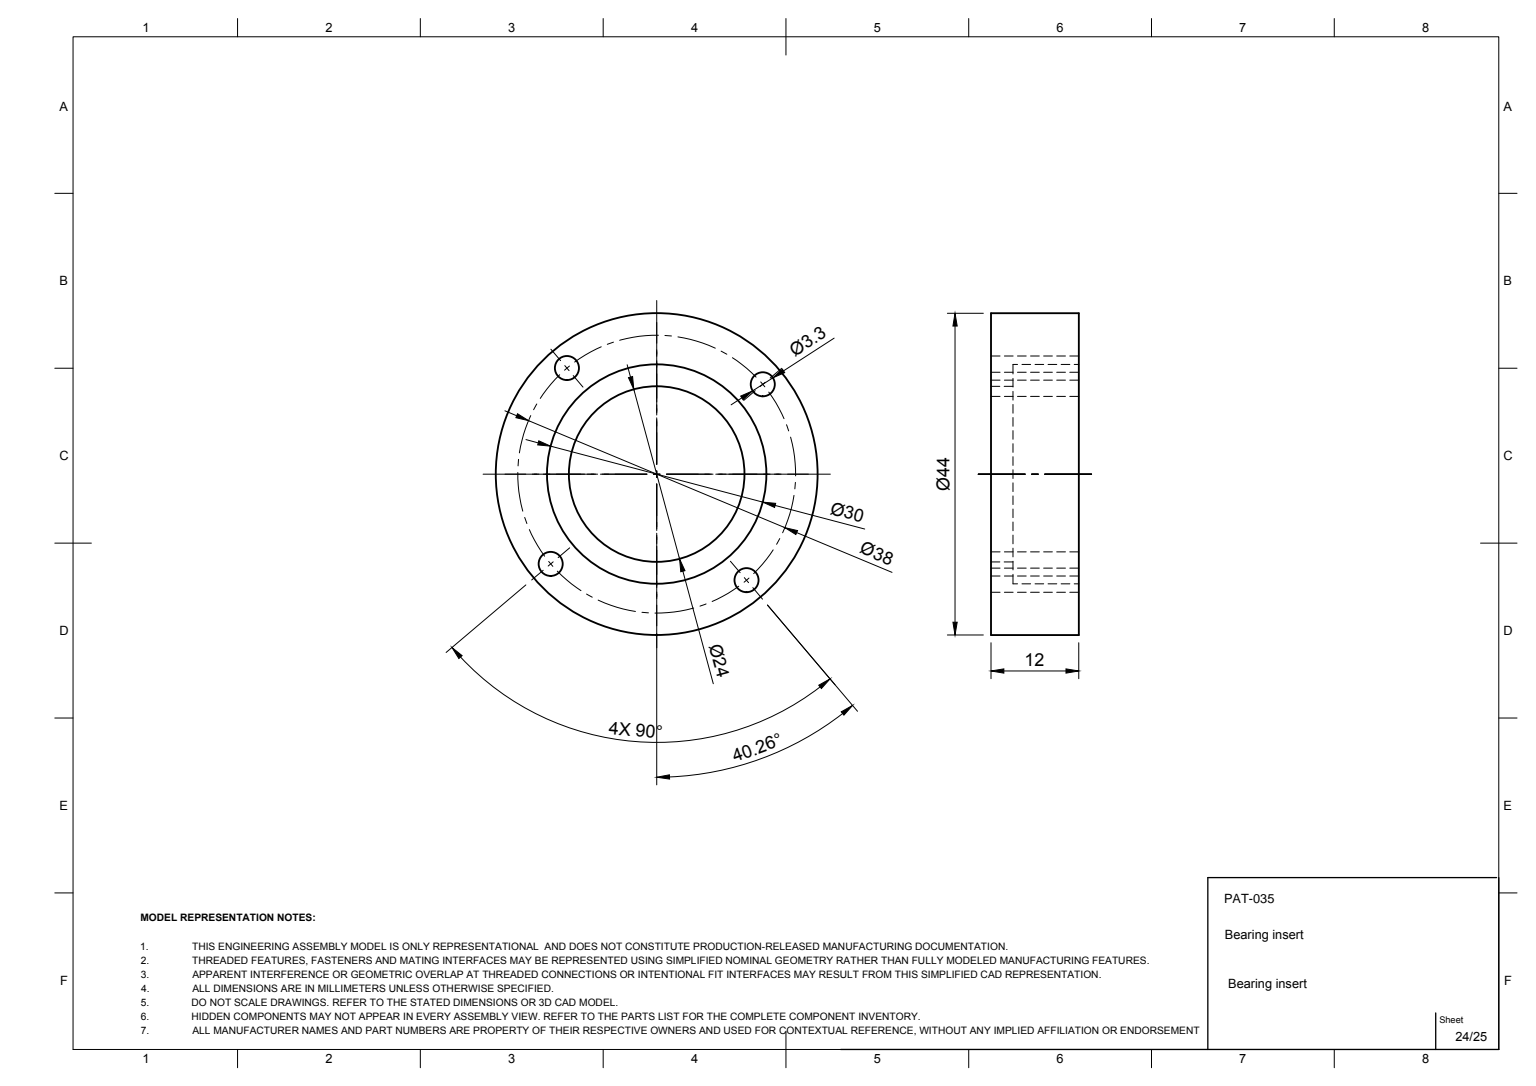
ISO-10303-21;
HEADER;
/* Generated by software containing ST-Developer
 * from STEP Tools, Inc. (www.steptools.com) 
 */

FILE_DESCRIPTION(
/* description */ ('Five-roller gravity conveyor'),
/* implementation_level */ '2;1');

FILE_NAME(
/* name */ 'Bearing insert.step',
/* time_stamp */ '2026-10-29T15:36:43-07:00',
/* author */ (''),
/* organization */ (''),
/* preprocessor_version */ 'ST-DEVELOPER v20.2',
/* originating_system */ 'Autodesk Translation Framework v15.17.0.0',
/* authorisation */ '');

FILE_SCHEMA (('AUTOMOTIVE_DESIGN { 1 0 10303 214 3 1 1 }'));
ENDSEC;

DATA;
#10=MECHANICAL_DESIGN_GEOMETRIC_PRESENTATION_REPRESENTATION('',(#335),#7806);
#291=SHAPE_REPRESENTATION_RELATIONSHIP('SRR','None',#7930,#309);
#309=ADVANCED_BREP_SHAPE_REPRESENTATION('',(#360),#7803);
#335=STYLED_ITEM('',(#8091),#360);
#360=MANIFOLD_SOLID_BREP('Body1',#4223);
#399=FACE_BOUND('',#1124,.T.);
#400=FACE_BOUND('',#1128,.T.);
#401=FACE_BOUND('',#1129,.T.);
#402=FACE_BOUND('',#1130,.T.);
#403=FACE_BOUND('',#1131,.T.);
#404=FACE_BOUND('',#1132,.T.);
#405=FACE_BOUND('',#1134,.T.);
#406=FACE_BOUND('',#1135,.T.);
#407=FACE_BOUND('',#1136,.T.);
#408=FACE_BOUND('',#1137,.T.);
#409=FACE_BOUND('',#1138,.T.);
#560=CIRCLE('',#4791,0.165);
#561=CIRCLE('',#4792,0.165);
#562=CIRCLE('',#4794,0.165);
#563=CIRCLE('',#4795,0.165);
#564=CIRCLE('',#4797,0.165);
#565=CIRCLE('',#4798,0.165);
#566=CIRCLE('',#4800,0.165);
#567=CIRCLE('',#4801,0.165);
#568=CIRCLE('',#4803,1.2);
#569=CIRCLE('',#4804,1.2);
#570=CIRCLE('',#4806,1.5);
#571=CIRCLE('',#4808,1.5);
#572=CIRCLE('',#4810,2.2);
#573=CIRCLE('',#4811,2.2);
#637=CYLINDRICAL_SURFACE('',#4790,0.165);
#638=CYLINDRICAL_SURFACE('',#4793,0.165);
#639=CYLINDRICAL_SURFACE('',#4796,0.165);
#640=CYLINDRICAL_SURFACE('',#4799,0.165);
#641=CYLINDRICAL_SURFACE('',#4802,1.2);
#642=CYLINDRICAL_SURFACE('',#4807,1.5);
#643=CYLINDRICAL_SURFACE('',#4809,2.2);
#849=FACE_OUTER_BOUND('',#1118,.T.);
#850=FACE_OUTER_BOUND('',#1119,.T.);
#851=FACE_OUTER_BOUND('',#1120,.T.);
#852=FACE_OUTER_BOUND('',#1121,.T.);
#853=FACE_OUTER_BOUND('',#1122,.T.);
#854=FACE_OUTER_BOUND('',#1123,.T.);
#855=FACE_OUTER_BOUND('',#1125,.T.);
#856=FACE_OUTER_BOUND('',#1126,.T.);
#857=FACE_OUTER_BOUND('',#1127,.T.);
#858=FACE_OUTER_BOUND('',#1133,.T.);
#1118=EDGE_LOOP('',(#3680,#3681,#3682,#3683));
#1119=EDGE_LOOP('',(#3684,#3685,#3686,#3687));
#1120=EDGE_LOOP('',(#3688,#3689,#3690,#3691));
#1121=EDGE_LOOP('',(#3692,#3693,#3694,#3695));
#1122=EDGE_LOOP('',(#3696,#3697,#3698,#3699));
#1123=EDGE_LOOP('',(#3700));
#1124=EDGE_LOOP('',(#3701));
#1125=EDGE_LOOP('',(#3702,#3703,#3704,#3705));
#1126=EDGE_LOOP('',(#3706,#3707,#3708,#3709));
#1127=EDGE_LOOP('',(#3710));
#1128=EDGE_LOOP('',(#3711));
#1129=EDGE_LOOP('',(#3712));
#1130=EDGE_LOOP('',(#3713));
#1131=EDGE_LOOP('',(#3714));
#1132=EDGE_LOOP('',(#3715));
#1133=EDGE_LOOP('',(#3716));
#1134=EDGE_LOOP('',(#3717));
#1135=EDGE_LOOP('',(#3718));
#1136=EDGE_LOOP('',(#3719));
#1137=EDGE_LOOP('',(#3720));
#1138=EDGE_LOOP('',(#3721));
#1479=LINE('',#7561,#1820);
#1480=LINE('',#7567,#1821);
#1481=LINE('',#7573,#1822);
#1482=LINE('',#7579,#1823);
#1483=LINE('',#7585,#1824);
#1484=LINE('',#7592,#1825);
#1485=LINE('',#7598,#1826);
#1820=VECTOR('',#5945,0.165);
#1821=VECTOR('',#5952,0.165);
#1822=VECTOR('',#5959,0.165);
#1823=VECTOR('',#5966,0.165);
#1824=VECTOR('',#5973,1.2);
#1825=VECTOR('',#5982,1.5);
#1826=VECTOR('',#5989,2.2);
#2174=VERTEX_POINT('',#7558);
#2175=VERTEX_POINT('',#7560);
#2176=VERTEX_POINT('',#7564);
#2177=VERTEX_POINT('',#7566);
#2178=VERTEX_POINT('',#7570);
#2179=VERTEX_POINT('',#7572);
#2180=VERTEX_POINT('',#7576);
#2181=VERTEX_POINT('',#7578);
#2182=VERTEX_POINT('',#7582);
#2183=VERTEX_POINT('',#7584);
#2184=VERTEX_POINT('',#7588);
#2185=VERTEX_POINT('',#7591);
#2186=VERTEX_POINT('',#7595);
#2187=VERTEX_POINT('',#7597);
#2683=EDGE_CURVE('',#2174,#2174,#560,.T.);
#2684=EDGE_CURVE('',#2174,#2175,#1479,.T.);
#2685=EDGE_CURVE('',#2175,#2175,#561,.T.);
#2686=EDGE_CURVE('',#2176,#2176,#562,.T.);
#2687=EDGE_CURVE('',#2176,#2177,#1480,.T.);
#2688=EDGE_CURVE('',#2177,#2177,#563,.T.);
#2689=EDGE_CURVE('',#2178,#2178,#564,.T.);
#2690=EDGE_CURVE('',#2178,#2179,#1481,.T.);
#2691=EDGE_CURVE('',#2179,#2179,#565,.T.);
#2692=EDGE_CURVE('',#2180,#2180,#566,.T.);
#2693=EDGE_CURVE('',#2180,#2181,#1482,.T.);
#2694=EDGE_CURVE('',#2181,#2181,#567,.T.);
#2695=EDGE_CURVE('',#2182,#2182,#568,.T.);
#2696=EDGE_CURVE('',#2182,#2183,#1483,.T.);
#2697=EDGE_CURVE('',#2183,#2183,#569,.T.);
#2698=EDGE_CURVE('',#2184,#2184,#570,.T.);
#2699=EDGE_CURVE('',#2184,#2185,#1484,.T.);
#2700=EDGE_CURVE('',#2185,#2185,#571,.T.);
#2701=EDGE_CURVE('',#2186,#2186,#572,.T.);
#2702=EDGE_CURVE('',#2186,#2187,#1485,.T.);
#2703=EDGE_CURVE('',#2187,#2187,#573,.T.);
#3680=ORIENTED_EDGE('',*,*,#2683,.F.);
#3681=ORIENTED_EDGE('',*,*,#2684,.T.);
#3682=ORIENTED_EDGE('',*,*,#2685,.F.);
#3683=ORIENTED_EDGE('',*,*,#2684,.F.);
#3684=ORIENTED_EDGE('',*,*,#2686,.F.);
#3685=ORIENTED_EDGE('',*,*,#2687,.T.);
#3686=ORIENTED_EDGE('',*,*,#2688,.F.);
#3687=ORIENTED_EDGE('',*,*,#2687,.F.);
#3688=ORIENTED_EDGE('',*,*,#2689,.F.);
#3689=ORIENTED_EDGE('',*,*,#2690,.T.);
#3690=ORIENTED_EDGE('',*,*,#2691,.F.);
#3691=ORIENTED_EDGE('',*,*,#2690,.F.);
#3692=ORIENTED_EDGE('',*,*,#2692,.F.);
#3693=ORIENTED_EDGE('',*,*,#2693,.T.);
#3694=ORIENTED_EDGE('',*,*,#2694,.F.);
#3695=ORIENTED_EDGE('',*,*,#2693,.F.);
#3696=ORIENTED_EDGE('',*,*,#2695,.F.);
#3697=ORIENTED_EDGE('',*,*,#2696,.T.);
#3698=ORIENTED_EDGE('',*,*,#2697,.T.);
#3699=ORIENTED_EDGE('',*,*,#2696,.F.);
#3700=ORIENTED_EDGE('',*,*,#2698,.F.);
#3701=ORIENTED_EDGE('',*,*,#2697,.F.);
#3702=ORIENTED_EDGE('',*,*,#2698,.T.);
#3703=ORIENTED_EDGE('',*,*,#2699,.T.);
#3704=ORIENTED_EDGE('',*,*,#2700,.T.);
#3705=ORIENTED_EDGE('',*,*,#2699,.F.);
#3706=ORIENTED_EDGE('',*,*,#2701,.F.);
#3707=ORIENTED_EDGE('',*,*,#2702,.T.);
#3708=ORIENTED_EDGE('',*,*,#2703,.T.);
#3709=ORIENTED_EDGE('',*,*,#2702,.F.);
#3710=ORIENTED_EDGE('',*,*,#2701,.T.);
#3711=ORIENTED_EDGE('',*,*,#2695,.T.);
#3712=ORIENTED_EDGE('',*,*,#2694,.T.);
#3713=ORIENTED_EDGE('',*,*,#2691,.T.);
#3714=ORIENTED_EDGE('',*,*,#2688,.T.);
#3715=ORIENTED_EDGE('',*,*,#2685,.T.);
#3716=ORIENTED_EDGE('',*,*,#2703,.F.);
#3717=ORIENTED_EDGE('',*,*,#2700,.F.);
#3718=ORIENTED_EDGE('',*,*,#2692,.T.);
#3719=ORIENTED_EDGE('',*,*,#2689,.T.);
#3720=ORIENTED_EDGE('',*,*,#2686,.T.);
#3721=ORIENTED_EDGE('',*,*,#2683,.T.);
#3951=PLANE('',#4805);
#3952=PLANE('',#4812);
#3953=PLANE('',#4813);
#4164=ADVANCED_FACE('',(#849),#637,.F.);
#4165=ADVANCED_FACE('',(#850),#638,.F.);
#4166=ADVANCED_FACE('',(#851),#639,.F.);
#4167=ADVANCED_FACE('',(#852),#640,.F.);
#4168=ADVANCED_FACE('',(#853),#641,.F.);
#4169=ADVANCED_FACE('',(#854,#399),#3951,.F.);
#4170=ADVANCED_FACE('',(#855),#642,.F.);
#4171=ADVANCED_FACE('',(#856),#643,.T.);
#4172=ADVANCED_FACE('',(#857,#400,#401,#402,#403,#404),#3952,.T.);
#4173=ADVANCED_FACE('',(#858,#405,#406,#407,#408,#409),#3953,.F.);
#4223=CLOSED_SHELL('',(#4164,#4165,#4166,#4167,#4168,#4169,#4170,#4171,
#4172,#4173));
#4789=AXIS2_PLACEMENT_3D('',#7556,#5939,#5940);
#4790=AXIS2_PLACEMENT_3D('',#7557,#5941,#5942);
#4791=AXIS2_PLACEMENT_3D('',#7559,#5943,#5944);
#4792=AXIS2_PLACEMENT_3D('',#7562,#5946,#5947);
#4793=AXIS2_PLACEMENT_3D('',#7563,#5948,#5949);
#4794=AXIS2_PLACEMENT_3D('',#7565,#5950,#5951);
#4795=AXIS2_PLACEMENT_3D('',#7568,#5953,#5954);
#4796=AXIS2_PLACEMENT_3D('',#7569,#5955,#5956);
#4797=AXIS2_PLACEMENT_3D('',#7571,#5957,#5958);
#4798=AXIS2_PLACEMENT_3D('',#7574,#5960,#5961);
#4799=AXIS2_PLACEMENT_3D('',#7575,#5962,#5963);
#4800=AXIS2_PLACEMENT_3D('',#7577,#5964,#5965);
#4801=AXIS2_PLACEMENT_3D('',#7580,#5967,#5968);
#4802=AXIS2_PLACEMENT_3D('',#7581,#5969,#5970);
#4803=AXIS2_PLACEMENT_3D('',#7583,#5971,#5972);
#4804=AXIS2_PLACEMENT_3D('',#7586,#5974,#5975);
#4805=AXIS2_PLACEMENT_3D('',#7587,#5976,#5977);
#4806=AXIS2_PLACEMENT_3D('',#7589,#5978,#5979);
#4807=AXIS2_PLACEMENT_3D('',#7590,#5980,#5981);
#4808=AXIS2_PLACEMENT_3D('',#7593,#5983,#5984);
#4809=AXIS2_PLACEMENT_3D('',#7594,#5985,#5986);
#4810=AXIS2_PLACEMENT_3D('',#7596,#5987,#5988);
#4811=AXIS2_PLACEMENT_3D('',#7599,#5990,#5991);
#4812=AXIS2_PLACEMENT_3D('',#7600,#5992,#5993);
#4813=AXIS2_PLACEMENT_3D('',#7601,#5994,#5995);
#5939=DIRECTION('axis',(0.,0.,1.));
#5940=DIRECTION('refdir',(1.,0.,0.));
#5941=DIRECTION('center_axis',(0.,1.,0.));
#5942=DIRECTION('ref_axis',(1.,0.,0.));
#5943=DIRECTION('center_axis',(0.,1.,0.));
#5944=DIRECTION('ref_axis',(1.,0.,0.));
#5945=DIRECTION('',(0.,1.,0.));
#5946=DIRECTION('center_axis',(0.,-1.,0.));
#5947=DIRECTION('ref_axis',(1.,0.,0.));
#5948=DIRECTION('center_axis',(0.,1.,0.));
#5949=DIRECTION('ref_axis',(1.,0.,0.));
#5950=DIRECTION('center_axis',(0.,1.,0.));
#5951=DIRECTION('ref_axis',(1.,0.,0.));
#5952=DIRECTION('',(0.,1.,0.));
#5953=DIRECTION('center_axis',(0.,-1.,0.));
#5954=DIRECTION('ref_axis',(1.,0.,0.));
#5955=DIRECTION('center_axis',(0.,1.,0.));
#5956=DIRECTION('ref_axis',(1.,0.,0.));
#5957=DIRECTION('center_axis',(0.,1.,0.));
#5958=DIRECTION('ref_axis',(1.,0.,0.));
#5959=DIRECTION('',(0.,1.,0.));
#5960=DIRECTION('center_axis',(0.,-1.,0.));
#5961=DIRECTION('ref_axis',(1.,0.,0.));
#5962=DIRECTION('center_axis',(0.,1.,0.));
#5963=DIRECTION('ref_axis',(1.,0.,0.));
#5964=DIRECTION('center_axis',(0.,1.,0.));
#5965=DIRECTION('ref_axis',(1.,0.,0.));
#5966=DIRECTION('',(0.,1.,0.));
#5967=DIRECTION('center_axis',(0.,-1.,0.));
#5968=DIRECTION('ref_axis',(1.,0.,0.));
#5969=DIRECTION('center_axis',(0.,1.,0.));
#5970=DIRECTION('ref_axis',(1.,0.,0.));
#5971=DIRECTION('center_axis',(0.,-1.,0.));
#5972=DIRECTION('ref_axis',(1.,0.,0.));
#5973=DIRECTION('',(0.,-1.,0.));
#5974=DIRECTION('center_axis',(0.,-1.,0.));
#5975=DIRECTION('ref_axis',(1.,0.,0.));
#5976=DIRECTION('center_axis',(0.,1.,0.));
#5977=DIRECTION('ref_axis',(1.,0.,0.));
#5978=DIRECTION('center_axis',(0.,1.,0.));
#5979=DIRECTION('ref_axis',(1.,0.,0.));
#5980=DIRECTION('center_axis',(0.,1.,0.));
#5981=DIRECTION('ref_axis',(1.,0.,0.));
#5982=DIRECTION('',(0.,-1.,0.));
#5983=DIRECTION('center_axis',(0.,-1.,0.));
#5984=DIRECTION('ref_axis',(1.,0.,0.));
#5985=DIRECTION('center_axis',(0.,1.,0.));
#5986=DIRECTION('ref_axis',(1.,0.,0.));
#5987=DIRECTION('center_axis',(0.,1.,0.));
#5988=DIRECTION('ref_axis',(1.,0.,0.));
#5989=DIRECTION('',(0.,-1.,0.));
#5990=DIRECTION('center_axis',(0.,1.,0.));
#5991=DIRECTION('ref_axis',(1.,0.,0.));
#5992=DIRECTION('center_axis',(0.,1.,0.));
#5993=DIRECTION('ref_axis',(1.,0.,0.));
#5994=DIRECTION('center_axis',(0.,1.,0.));
#5995=DIRECTION('ref_axis',(1.,0.,0.));
#7556=CARTESIAN_POINT('',(0.,0.,0.));
#7557=CARTESIAN_POINT('Origin',(-1.9,-0.1,4.5));
#7558=CARTESIAN_POINT('',(-2.065,0.,4.5));
#7559=CARTESIAN_POINT('Origin',(-1.9,0.,4.5));
#7560=CARTESIAN_POINT('',(-2.065,1.2,4.5));
#7561=CARTESIAN_POINT('',(-2.065,-0.1,4.5));
#7562=CARTESIAN_POINT('Origin',(-1.9,1.2,4.5));
#7563=CARTESIAN_POINT('Origin',(1.16341445918999E-16,-0.1,6.4));
#7564=CARTESIAN_POINT('',(-0.165,0.,6.4));
#7565=CARTESIAN_POINT('Origin',(1.16341445918999E-16,0.,6.4));
#7566=CARTESIAN_POINT('',(-0.165,1.2,6.4));
#7567=CARTESIAN_POINT('',(-0.165,-0.1,6.4));
#7568=CARTESIAN_POINT('Origin',(1.16341445918999E-16,1.2,6.4));
#7569=CARTESIAN_POINT('Origin',(1.9,-0.1,4.5));
#7570=CARTESIAN_POINT('',(1.735,0.,4.5));
#7571=CARTESIAN_POINT('Origin',(1.9,0.,4.5));
#7572=CARTESIAN_POINT('',(1.735,1.2,4.5));
#7573=CARTESIAN_POINT('',(1.735,-0.1,4.5));
#7574=CARTESIAN_POINT('Origin',(1.9,1.2,4.5));
#7575=CARTESIAN_POINT('Origin',(-3.49024337756996E-16,-0.1,2.6));
#7576=CARTESIAN_POINT('',(-0.165,0.,2.6));
#7577=CARTESIAN_POINT('Origin',(-3.49024337756996E-16,0.,2.6));
#7578=CARTESIAN_POINT('',(-0.165,1.2,2.6));
#7579=CARTESIAN_POINT('',(-0.165,-0.1,2.6));
#7580=CARTESIAN_POINT('Origin',(-3.49024337756996E-16,1.2,2.6));
#7581=CARTESIAN_POINT('Origin',(0.,0.9,4.5));
#7582=CARTESIAN_POINT('',(-1.2,1.2,4.5));
#7583=CARTESIAN_POINT('Origin',(0.,1.2,4.5));
#7584=CARTESIAN_POINT('',(-1.2,0.9,4.5));
#7585=CARTESIAN_POINT('',(-1.2,0.9,4.5));
#7586=CARTESIAN_POINT('Origin',(0.,0.9,4.5));
#7587=CARTESIAN_POINT('Origin',(0.,0.9,4.5));
#7588=CARTESIAN_POINT('',(-1.5,0.9,4.5));
#7589=CARTESIAN_POINT('Origin',(0.,0.9,4.5));
#7590=CARTESIAN_POINT('Origin',(0.,0.,4.5));
#7591=CARTESIAN_POINT('',(-1.5,0.,4.5));
#7592=CARTESIAN_POINT('',(-1.5,0.,4.5));
#7593=CARTESIAN_POINT('Origin',(0.,0.,4.5));
#7594=CARTESIAN_POINT('Origin',(0.,0.,4.5));
#7595=CARTESIAN_POINT('',(-2.2,1.2,4.5));
#7596=CARTESIAN_POINT('Origin',(0.,1.2,4.5));
#7597=CARTESIAN_POINT('',(-2.2,0.,4.5));
#7598=CARTESIAN_POINT('',(-2.2,0.,4.5));
#7599=CARTESIAN_POINT('Origin',(0.,0.,4.5));
#7600=CARTESIAN_POINT('Origin',(0.,1.2,4.5));
#7601=CARTESIAN_POINT('Origin',(0.,0.,4.5));
#7779=UNCERTAINTY_MEASURE_WITH_UNIT(LENGTH_MEASURE(0.001),#7807,
'DISTANCE_ACCURACY_VALUE',
'Maximum model space distance between geometric entities at asserted c
onnectivities');
#7782=UNCERTAINTY_MEASURE_WITH_UNIT(LENGTH_MEASURE(0.001),#7807,
'DISTANCE_ACCURACY_VALUE',
'Maximum model space distance between geometric entities at asserted c
onnectivities');
#7803=(
GEOMETRIC_REPRESENTATION_CONTEXT(3)
GLOBAL_UNCERTAINTY_ASSIGNED_CONTEXT((#7779))
GLOBAL_UNIT_ASSIGNED_CONTEXT((#7807,#7809,#7810))
REPRESENTATION_CONTEXT('','3D')
);
#7806=(
GEOMETRIC_REPRESENTATION_CONTEXT(3)
GLOBAL_UNCERTAINTY_ASSIGNED_CONTEXT((#7782))
GLOBAL_UNIT_ASSIGNED_CONTEXT((#7807,#7809,#7810))
REPRESENTATION_CONTEXT('','3D')
);
#7807=(
LENGTH_UNIT()
NAMED_UNIT(*)
SI_UNIT(.CENTI.,.METRE.)
);
#7809=(
NAMED_UNIT(*)
PLANE_ANGLE_UNIT()
SI_UNIT($,.RADIAN.)
);
#7810=(
NAMED_UNIT(*)
SI_UNIT($,.STERADIAN.)
SOLID_ANGLE_UNIT()
);
#7831=SHAPE_DEFINITION_REPRESENTATION(#7859,#7930);
#7859=PRODUCT_DEFINITION_SHAPE('',$,#7954);
#7930=SHAPE_REPRESENTATION('',(#4789),#7803);
#7933=PRODUCT_DEFINITION_CONTEXT('part definition',#8004,'design');
#7954=PRODUCT_DEFINITION('Bearing insert','Bearing insert',#7977,#7933);
#7977=PRODUCT_DEFINITION_FORMATION('',$,#8026);
#8004=APPLICATION_CONTEXT(
'Core Data for Automotive Mechanical Design Process');
#8005=PRODUCT_CONTEXT('part definition',#8004,'mechanical');
#8026=PRODUCT('Bearing insert','Bearing insert','Bearing insert',(#8005));
#8085=COLOUR_RGB('Grey',0.48,0.52,0.57);
#8086=FILL_AREA_STYLE_COLOUR('',#8085);
#8087=FILL_AREA_STYLE('',(#8086));
#8088=SURFACE_STYLE_FILL_AREA(#8087);
#8089=SURFACE_SIDE_STYLE('',(#8088));
#8090=SURFACE_STYLE_USAGE(.BOTH.,#8089);
#8091=PRESENTATION_STYLE_ASSIGNMENT((#8090));
ENDSEC;
END-ISO-10303-21;
